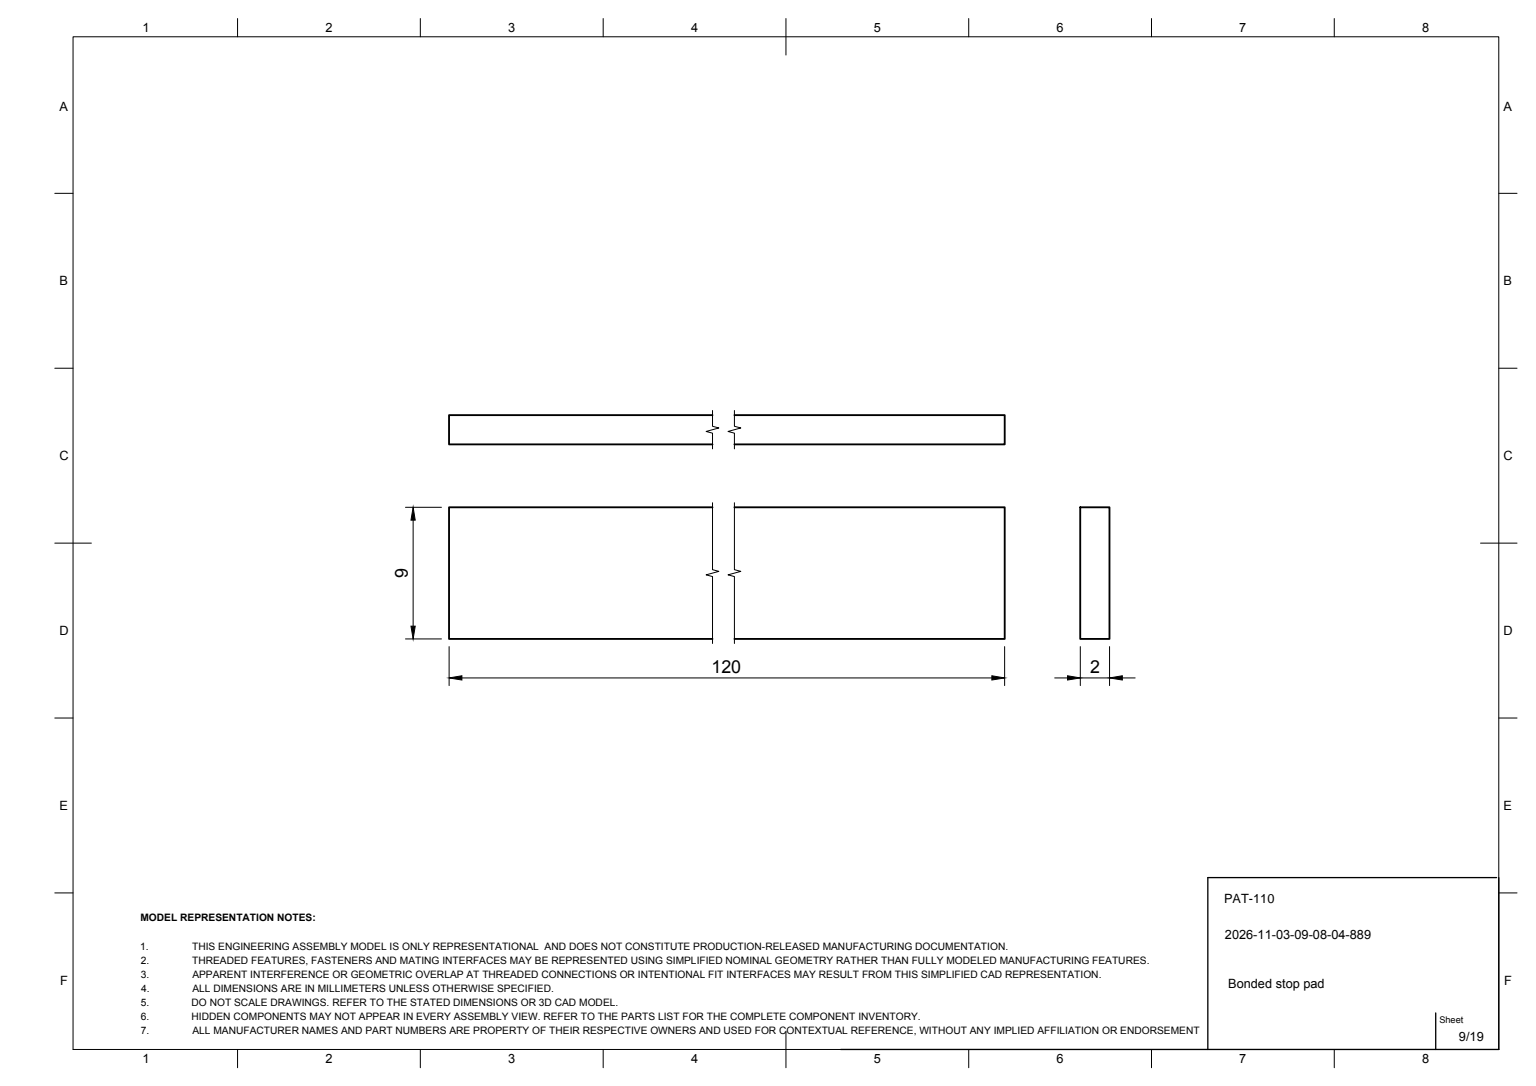
ISO-10303-21;
HEADER;
/* Generated by software containing ST-Developer
 * from STEP Tools, Inc. (www.steptools.com) 
 */

FILE_DESCRIPTION(
/* description */ ('Twin-shaft manual slide'),
/* implementation_level */ '2;1');

FILE_NAME(
/* name */ 'Bonded stop pad.step',
/* time_stamp */ '2026-10-27T18:38:08-07:00',
/* author */ (''),
/* organization */ (''),
/* preprocessor_version */ 'ST-DEVELOPER v20.2',
/* originating_system */ 'Autodesk Translation Framework v15.17.0.0',
/* authorisation */ '');

FILE_SCHEMA (('AUTOMOTIVE_DESIGN { 1 0 10303 214 3 1 1 }'));
ENDSEC;

DATA;
#10=MECHANICAL_DESIGN_GEOMETRIC_PRESENTATION_REPRESENTATION('',(#281),#6463);
#249=SHAPE_REPRESENTATION_RELATIONSHIP('SRR','None',#6567,#265);
#265=ADVANCED_BREP_SHAPE_REPRESENTATION('',(#296),#6450);
#281=STYLED_ITEM('',(#6754),#296);
#296=MANIFOLD_SOLID_BREP('Body1',#3644);
#444=PLANE('',#3974);
#445=PLANE('',#3975);
#446=PLANE('',#3976);
#447=PLANE('',#3977);
#448=PLANE('',#3978);
#449=PLANE('',#3979);
#600=FACE_OUTER_BOUND('',#848,.T.);
#601=FACE_OUTER_BOUND('',#849,.T.);
#602=FACE_OUTER_BOUND('',#850,.T.);
#603=FACE_OUTER_BOUND('',#851,.T.);
#604=FACE_OUTER_BOUND('',#852,.T.);
#605=FACE_OUTER_BOUND('',#853,.T.);
#848=EDGE_LOOP('',(#2832,#2833,#2834,#2835));
#849=EDGE_LOOP('',(#2836,#2837,#2838,#2839));
#850=EDGE_LOOP('',(#2840,#2841,#2842,#2843));
#851=EDGE_LOOP('',(#2844,#2845,#2846,#2847));
#852=EDGE_LOOP('',(#2848,#2849,#2850,#2851));
#853=EDGE_LOOP('',(#2852,#2853,#2854,#2855));
#1152=LINE('',#5787,#1438);
#1153=LINE('',#5789,#1439);
#1154=LINE('',#5791,#1440);
#1155=LINE('',#5792,#1441);
#1156=LINE('',#5795,#1442);
#1157=LINE('',#5797,#1443);
#1158=LINE('',#5798,#1444);
#1159=LINE('',#5801,#1445);
#1160=LINE('',#5803,#1446);
#1161=LINE('',#5804,#1447);
#1162=LINE('',#5806,#1448);
#1163=LINE('',#5807,#1449);
#1438=VECTOR('',#4662,1.);
#1439=VECTOR('',#4663,1.);
#1440=VECTOR('',#4664,1.);
#1441=VECTOR('',#4665,1.);
#1442=VECTOR('',#4668,1.);
#1443=VECTOR('',#4669,1.);
#1444=VECTOR('',#4670,1.);
#1445=VECTOR('',#4673,1.);
#1446=VECTOR('',#4674,1.);
#1447=VECTOR('',#4675,1.);
#1448=VECTOR('',#4678,1.);
#1449=VECTOR('',#4679,1.);
#1875=VERTEX_POINT('',#5785);
#1876=VERTEX_POINT('',#5786);
#1877=VERTEX_POINT('',#5788);
#1878=VERTEX_POINT('',#5790);
#1879=VERTEX_POINT('',#5794);
#1880=VERTEX_POINT('',#5796);
#1881=VERTEX_POINT('',#5800);
#1882=VERTEX_POINT('',#5802);
#2221=EDGE_CURVE('',#1875,#1876,#1152,.T.);
#2222=EDGE_CURVE('',#1876,#1877,#1153,.T.);
#2223=EDGE_CURVE('',#1878,#1877,#1154,.T.);
#2224=EDGE_CURVE('',#1875,#1878,#1155,.T.);
#2225=EDGE_CURVE('',#1879,#1875,#1156,.T.);
#2226=EDGE_CURVE('',#1880,#1878,#1157,.T.);
#2227=EDGE_CURVE('',#1879,#1880,#1158,.T.);
#2228=EDGE_CURVE('',#1881,#1879,#1159,.T.);
#2229=EDGE_CURVE('',#1882,#1880,#1160,.T.);
#2230=EDGE_CURVE('',#1881,#1882,#1161,.T.);
#2231=EDGE_CURVE('',#1876,#1881,#1162,.T.);
#2232=EDGE_CURVE('',#1877,#1882,#1163,.T.);
#2832=ORIENTED_EDGE('',*,*,#2221,.T.);
#2833=ORIENTED_EDGE('',*,*,#2222,.T.);
#2834=ORIENTED_EDGE('',*,*,#2223,.F.);
#2835=ORIENTED_EDGE('',*,*,#2224,.F.);
#2836=ORIENTED_EDGE('',*,*,#2225,.T.);
#2837=ORIENTED_EDGE('',*,*,#2224,.T.);
#2838=ORIENTED_EDGE('',*,*,#2226,.F.);
#2839=ORIENTED_EDGE('',*,*,#2227,.F.);
#2840=ORIENTED_EDGE('',*,*,#2228,.T.);
#2841=ORIENTED_EDGE('',*,*,#2227,.T.);
#2842=ORIENTED_EDGE('',*,*,#2229,.F.);
#2843=ORIENTED_EDGE('',*,*,#2230,.F.);
#2844=ORIENTED_EDGE('',*,*,#2231,.T.);
#2845=ORIENTED_EDGE('',*,*,#2230,.T.);
#2846=ORIENTED_EDGE('',*,*,#2232,.F.);
#2847=ORIENTED_EDGE('',*,*,#2222,.F.);
#2848=ORIENTED_EDGE('',*,*,#2232,.T.);
#2849=ORIENTED_EDGE('',*,*,#2229,.T.);
#2850=ORIENTED_EDGE('',*,*,#2226,.T.);
#2851=ORIENTED_EDGE('',*,*,#2223,.T.);
#2852=ORIENTED_EDGE('',*,*,#2231,.F.);
#2853=ORIENTED_EDGE('',*,*,#2221,.F.);
#2854=ORIENTED_EDGE('',*,*,#2225,.F.);
#2855=ORIENTED_EDGE('',*,*,#2228,.F.);
#3505=ADVANCED_FACE('',(#600),#444,.T.);
#3506=ADVANCED_FACE('',(#601),#445,.T.);
#3507=ADVANCED_FACE('',(#602),#446,.T.);
#3508=ADVANCED_FACE('',(#603),#447,.T.);
#3509=ADVANCED_FACE('',(#604),#448,.T.);
#3510=ADVANCED_FACE('',(#605),#449,.F.);
#3644=CLOSED_SHELL('',(#3505,#3506,#3507,#3508,#3509,#3510));
#3973=AXIS2_PLACEMENT_3D('',#5783,#4658,#4659);
#3974=AXIS2_PLACEMENT_3D('',#5784,#4660,#4661);
#3975=AXIS2_PLACEMENT_3D('',#5793,#4666,#4667);
#3976=AXIS2_PLACEMENT_3D('',#5799,#4671,#4672);
#3977=AXIS2_PLACEMENT_3D('',#5805,#4676,#4677);
#3978=AXIS2_PLACEMENT_3D('',#5808,#4680,#4681);
#3979=AXIS2_PLACEMENT_3D('',#5809,#4682,#4683);
#4658=DIRECTION('axis',(0.,0.,1.));
#4659=DIRECTION('refdir',(1.,0.,0.));
#4660=DIRECTION('center_axis',(0.,1.,0.));
#4661=DIRECTION('ref_axis',(-1.,0.,0.));
#4662=DIRECTION('',(-1.,0.,0.));
#4663=DIRECTION('',(0.,0.,1.));
#4664=DIRECTION('',(-1.,0.,0.));
#4665=DIRECTION('',(0.,0.,1.));
#4666=DIRECTION('center_axis',(1.,0.,0.));
#4667=DIRECTION('ref_axis',(0.,1.,0.));
#4668=DIRECTION('',(0.,1.,0.));
#4669=DIRECTION('',(0.,1.,0.));
#4670=DIRECTION('',(0.,0.,1.));
#4671=DIRECTION('center_axis',(0.,-1.,0.));
#4672=DIRECTION('ref_axis',(1.,0.,0.));
#4673=DIRECTION('',(1.,0.,0.));
#4674=DIRECTION('',(1.,0.,0.));
#4675=DIRECTION('',(0.,0.,1.));
#4676=DIRECTION('center_axis',(-1.,0.,0.));
#4677=DIRECTION('ref_axis',(0.,-1.,0.));
#4678=DIRECTION('',(0.,-1.,0.));
#4679=DIRECTION('',(0.,-1.,0.));
#4680=DIRECTION('center_axis',(0.,0.,1.));
#4681=DIRECTION('ref_axis',(1.,0.,0.));
#4682=DIRECTION('center_axis',(0.,0.,1.));
#4683=DIRECTION('ref_axis',(1.,0.,0.));
#5783=CARTESIAN_POINT('',(0.,0.,0.));
#5784=CARTESIAN_POINT('Origin',(4.2,6.,1.6));
#5785=CARTESIAN_POINT('',(4.2,6.,1.6));
#5786=CARTESIAN_POINT('',(4.,6.,1.6));
#5787=CARTESIAN_POINT('',(4.2,6.,1.6));
#5788=CARTESIAN_POINT('',(4.,6.,2.5));
#5789=CARTESIAN_POINT('',(4.,6.,1.6));
#5790=CARTESIAN_POINT('',(4.2,6.,2.5));
#5791=CARTESIAN_POINT('',(4.2,6.,2.5));
#5792=CARTESIAN_POINT('',(4.2,6.,1.6));
#5793=CARTESIAN_POINT('Origin',(4.2,-6.,1.6));
#5794=CARTESIAN_POINT('',(4.2,-6.,1.6));
#5795=CARTESIAN_POINT('',(4.2,-6.,1.6));
#5796=CARTESIAN_POINT('',(4.2,-6.,2.5));
#5797=CARTESIAN_POINT('',(4.2,-6.,2.5));
#5798=CARTESIAN_POINT('',(4.2,-6.,1.6));
#5799=CARTESIAN_POINT('Origin',(4.,-6.,1.6));
#5800=CARTESIAN_POINT('',(4.,-6.,1.6));
#5801=CARTESIAN_POINT('',(4.,-6.,1.6));
#5802=CARTESIAN_POINT('',(4.,-6.,2.5));
#5803=CARTESIAN_POINT('',(4.,-6.,2.5));
#5804=CARTESIAN_POINT('',(4.,-6.,1.6));
#5805=CARTESIAN_POINT('Origin',(4.,6.,1.6));
#5806=CARTESIAN_POINT('',(4.,6.,1.6));
#5807=CARTESIAN_POINT('',(4.,6.,2.5));
#5808=CARTESIAN_POINT('Origin',(4.1,0.,2.5));
#5809=CARTESIAN_POINT('Origin',(4.1,0.,1.6));
#6429=UNCERTAINTY_MEASURE_WITH_UNIT(LENGTH_MEASURE(0.001),#6464,
'DISTANCE_ACCURACY_VALUE',
'Maximum model space distance between geometric entities at asserted c
onnectivities');
#6442=UNCERTAINTY_MEASURE_WITH_UNIT(LENGTH_MEASURE(0.001),#6464,
'DISTANCE_ACCURACY_VALUE',
'Maximum model space distance between geometric entities at asserted c
onnectivities');
#6450=(
GEOMETRIC_REPRESENTATION_CONTEXT(3)
GLOBAL_UNCERTAINTY_ASSIGNED_CONTEXT((#6429))
GLOBAL_UNIT_ASSIGNED_CONTEXT((#6464,#6466,#6467))
REPRESENTATION_CONTEXT('','3D')
);
#6463=(
GEOMETRIC_REPRESENTATION_CONTEXT(3)
GLOBAL_UNCERTAINTY_ASSIGNED_CONTEXT((#6442))
GLOBAL_UNIT_ASSIGNED_CONTEXT((#6464,#6466,#6467))
REPRESENTATION_CONTEXT('','3D')
);
#6464=(
LENGTH_UNIT()
NAMED_UNIT(*)
SI_UNIT(.CENTI.,.METRE.)
);
#6466=(
NAMED_UNIT(*)
PLANE_ANGLE_UNIT()
SI_UNIT($,.RADIAN.)
);
#6467=(
NAMED_UNIT(*)
SI_UNIT($,.STERADIAN.)
SOLID_ANGLE_UNIT()
);
#6475=SHAPE_DEFINITION_REPRESENTATION(#6495,#6567);
#6495=PRODUCT_DEFINITION_SHAPE('',$,#6588);
#6567=SHAPE_REPRESENTATION('',(#3973),#6450);
#6580=PRODUCT_DEFINITION_CONTEXT('part definition',#6642,'design');
#6588=PRODUCT_DEFINITION('Bonded stop pad','Bonded stop pad',#6608,#6580);
#6608=PRODUCT_DEFINITION_FORMATION('',$,#6651);
#6642=APPLICATION_CONTEXT(
'Core Data for Automotive Mechanical Design Process');
#6643=PRODUCT_CONTEXT('part definition',#6642,'mechanical');
#6651=PRODUCT('Bonded stop pad','Bonded stop pad','Bonded stop pad',(#6643));
#6748=COLOUR_RGB('Off White',0.89,0.88,0.83);
#6749=FILL_AREA_STYLE_COLOUR('',#6748);
#6750=FILL_AREA_STYLE('',(#6749));
#6751=SURFACE_STYLE_FILL_AREA(#6750);
#6752=SURFACE_SIDE_STYLE('',(#6751));
#6753=SURFACE_STYLE_USAGE(.BOTH.,#6752);
#6754=PRESENTATION_STYLE_ASSIGNMENT((#6753));
ENDSEC;
END-ISO-10303-21;
